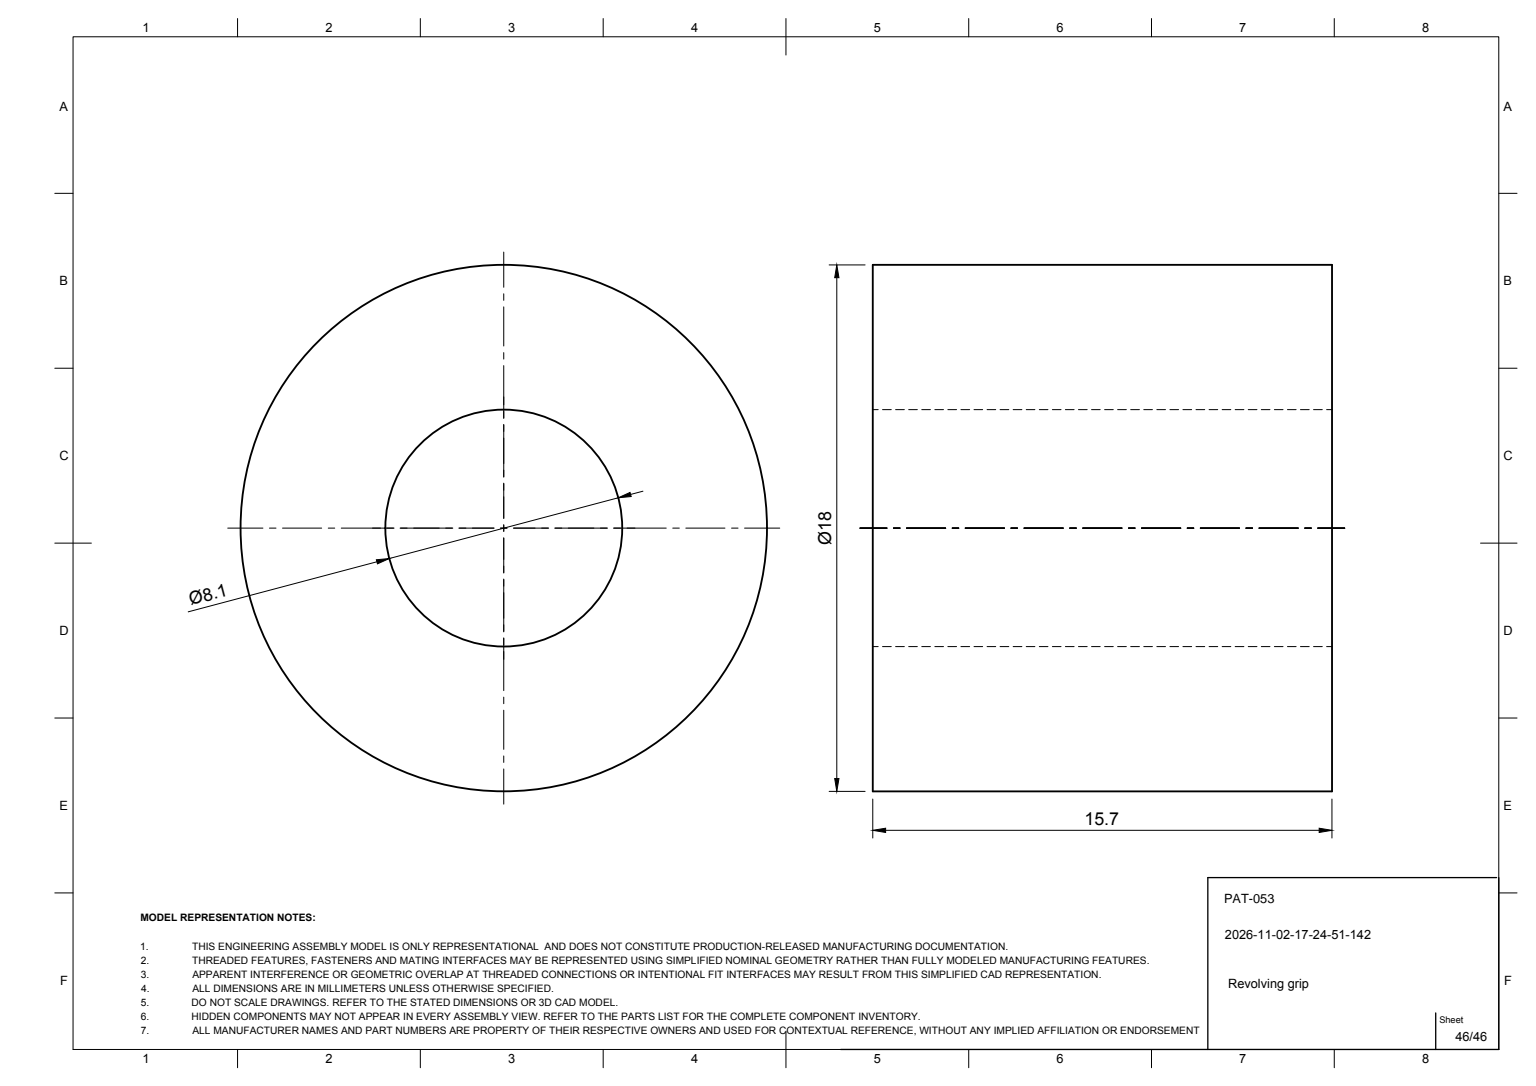
ISO-10303-21;
HEADER;
/* Generated by software containing ST-Developer
 * from STEP Tools, Inc. (www.steptools.com) 
 */

FILE_DESCRIPTION(
/* description */ ('Hand-operated arbor press'),
/* implementation_level */ '2;1');

FILE_NAME(
/* name */ 'Revolving grip.step',
/* time_stamp */ '2026-10-28T03:25:25-07:00',
/* author */ (''),
/* organization */ (''),
/* preprocessor_version */ 'ST-DEVELOPER v20.2',
/* originating_system */ 'Autodesk Translation Framework v15.17.0.0',
/* authorisation */ '');

FILE_SCHEMA (('AUTOMOTIVE_DESIGN { 1 0 10303 214 3 1 1 }'));
ENDSEC;

DATA;
#10=MECHANICAL_DESIGN_GEOMETRIC_PRESENTATION_REPRESENTATION('',(#634),#32751);
#543=SHAPE_REPRESENTATION_RELATIONSHIP('SRR','None',#32976,#585);
#585=ADVANCED_BREP_SHAPE_REPRESENTATION('',(#679),#32750);
#634=STYLED_ITEM('',(#33249),#679);
#679=MANIFOLD_SOLID_BREP('Body1',#12535);
#847=FACE_BOUND('',#2821,.T.);
#848=FACE_BOUND('',#2823,.T.);
#1291=PLANE('',#14148);
#1292=PLANE('',#14149);
#1970=FACE_OUTER_BOUND('',#2818,.T.);
#1971=FACE_OUTER_BOUND('',#2819,.T.);
#1972=FACE_OUTER_BOUND('',#2820,.T.);
#1973=FACE_OUTER_BOUND('',#2822,.T.);
#2818=EDGE_LOOP('',(#11630,#11631,#11632,#11633));
#2819=EDGE_LOOP('',(#11634,#11635,#11636,#11637));
#2820=EDGE_LOOP('',(#11638));
#2821=EDGE_LOOP('',(#11639));
#2822=EDGE_LOOP('',(#11640));
#2823=EDGE_LOOP('',(#11641));
#3993=LINE('',#32639,#5164);
#3994=LINE('',#32645,#5165);
#5164=VECTOR('',#17614,0.405);
#5165=VECTOR('',#17621,0.9);
#5552=CIRCLE('',#14143,0.405);
#5553=CIRCLE('',#14144,0.405);
#5554=CIRCLE('',#14146,0.9);
#5555=CIRCLE('',#14147,0.9);
#6661=VERTEX_POINT('',#32636);
#6662=VERTEX_POINT('',#32638);
#6663=VERTEX_POINT('',#32642);
#6664=VERTEX_POINT('',#32644);
#8318=EDGE_CURVE('',#6661,#6661,#5552,.T.);
#8319=EDGE_CURVE('',#6661,#6662,#3993,.T.);
#8320=EDGE_CURVE('',#6662,#6662,#5553,.T.);
#8321=EDGE_CURVE('',#6663,#6663,#5554,.T.);
#8322=EDGE_CURVE('',#6663,#6664,#3994,.T.);
#8323=EDGE_CURVE('',#6664,#6664,#5555,.T.);
#11630=ORIENTED_EDGE('',*,*,#8318,.F.);
#11631=ORIENTED_EDGE('',*,*,#8319,.T.);
#11632=ORIENTED_EDGE('',*,*,#8320,.T.);
#11633=ORIENTED_EDGE('',*,*,#8319,.F.);
#11634=ORIENTED_EDGE('',*,*,#8321,.F.);
#11635=ORIENTED_EDGE('',*,*,#8322,.T.);
#11636=ORIENTED_EDGE('',*,*,#8323,.T.);
#11637=ORIENTED_EDGE('',*,*,#8322,.F.);
#11638=ORIENTED_EDGE('',*,*,#8321,.T.);
#11639=ORIENTED_EDGE('',*,*,#8318,.T.);
#11640=ORIENTED_EDGE('',*,*,#8323,.F.);
#11641=ORIENTED_EDGE('',*,*,#8320,.F.);
#11800=CYLINDRICAL_SURFACE('',#14142,0.405);
#11801=CYLINDRICAL_SURFACE('',#14145,0.9);
#12479=ADVANCED_FACE('',(#1970),#11800,.F.);
#12480=ADVANCED_FACE('',(#1971),#11801,.T.);
#12481=ADVANCED_FACE('',(#1972,#847),#1291,.T.);
#12482=ADVANCED_FACE('',(#1973,#848),#1292,.F.);
#12535=CLOSED_SHELL('',(#12479,#12480,#12481,#12482));
#14141=AXIS2_PLACEMENT_3D('',#32634,#17608,#17609);
#14142=AXIS2_PLACEMENT_3D('',#32635,#17610,#17611);
#14143=AXIS2_PLACEMENT_3D('',#32637,#17612,#17613);
#14144=AXIS2_PLACEMENT_3D('',#32640,#17615,#17616);
#14145=AXIS2_PLACEMENT_3D('',#32641,#17617,#17618);
#14146=AXIS2_PLACEMENT_3D('',#32643,#17619,#17620);
#14147=AXIS2_PLACEMENT_3D('',#32646,#17622,#17623);
#14148=AXIS2_PLACEMENT_3D('',#32647,#17624,#17625);
#14149=AXIS2_PLACEMENT_3D('',#32648,#17626,#17627);
#17608=DIRECTION('axis',(0.,0.,1.));
#17609=DIRECTION('refdir',(1.,0.,0.));
#17610=DIRECTION('center_axis',(0.,1.,0.));
#17611=DIRECTION('ref_axis',(1.,0.,0.));
#17612=DIRECTION('center_axis',(0.,-1.,0.));
#17613=DIRECTION('ref_axis',(1.,0.,0.));
#17614=DIRECTION('',(0.,-1.,0.));
#17615=DIRECTION('center_axis',(0.,-1.,0.));
#17616=DIRECTION('ref_axis',(1.,0.,0.));
#17617=DIRECTION('center_axis',(0.,1.,0.));
#17618=DIRECTION('ref_axis',(1.,0.,0.));
#17619=DIRECTION('center_axis',(0.,1.,0.));
#17620=DIRECTION('ref_axis',(1.,0.,0.));
#17621=DIRECTION('',(0.,-1.,0.));
#17622=DIRECTION('center_axis',(0.,1.,0.));
#17623=DIRECTION('ref_axis',(1.,0.,0.));
#17624=DIRECTION('center_axis',(0.,1.,0.));
#17625=DIRECTION('ref_axis',(1.,0.,0.));
#17626=DIRECTION('center_axis',(0.,1.,0.));
#17627=DIRECTION('ref_axis',(1.,0.,0.));
#32634=CARTESIAN_POINT('',(0.,0.,0.));
#32635=CARTESIAN_POINT('Origin',(-3.25,6.8,29.));
#32636=CARTESIAN_POINT('',(-3.655,8.37,29.));
#32637=CARTESIAN_POINT('Origin',(-3.25,8.37,29.));
#32638=CARTESIAN_POINT('',(-3.655,6.8,29.));
#32639=CARTESIAN_POINT('',(-3.655,6.8,29.));
#32640=CARTESIAN_POINT('Origin',(-3.25,6.8,29.));
#32641=CARTESIAN_POINT('Origin',(-3.25,6.8,29.));
#32642=CARTESIAN_POINT('',(-4.15,8.37,29.));
#32643=CARTESIAN_POINT('Origin',(-3.25,8.37,29.));
#32644=CARTESIAN_POINT('',(-4.15,6.8,29.));
#32645=CARTESIAN_POINT('',(-4.15,6.8,29.));
#32646=CARTESIAN_POINT('Origin',(-3.25,6.8,29.));
#32647=CARTESIAN_POINT('Origin',(-3.25,8.37,29.));
#32648=CARTESIAN_POINT('Origin',(-3.25,6.8,29.));
#32701=UNCERTAINTY_MEASURE_WITH_UNIT(LENGTH_MEASURE(0.001),#32752,
'DISTANCE_ACCURACY_VALUE',
'Maximum model space distance between geometric entities at asserted c
onnectivities');
#32702=UNCERTAINTY_MEASURE_WITH_UNIT(LENGTH_MEASURE(0.001),#32752,
'DISTANCE_ACCURACY_VALUE',
'Maximum model space distance between geometric entities at asserted c
onnectivities');
#32750=(
GEOMETRIC_REPRESENTATION_CONTEXT(3)
GLOBAL_UNCERTAINTY_ASSIGNED_CONTEXT((#32701))
GLOBAL_UNIT_ASSIGNED_CONTEXT((#32752,#32754,#32755))
REPRESENTATION_CONTEXT('','3D')
);
#32751=(
GEOMETRIC_REPRESENTATION_CONTEXT(3)
GLOBAL_UNCERTAINTY_ASSIGNED_CONTEXT((#32702))
GLOBAL_UNIT_ASSIGNED_CONTEXT((#32752,#32754,#32755))
REPRESENTATION_CONTEXT('','3D')
);
#32752=(
LENGTH_UNIT()
NAMED_UNIT(*)
SI_UNIT(.CENTI.,.METRE.)
);
#32754=(
NAMED_UNIT(*)
PLANE_ANGLE_UNIT()
SI_UNIT($,.RADIAN.)
);
#32755=(
NAMED_UNIT(*)
SI_UNIT($,.STERADIAN.)
SOLID_ANGLE_UNIT()
);
#32803=SHAPE_DEFINITION_REPRESENTATION(#32923,#32976);
#32923=PRODUCT_DEFINITION_SHAPE('',$,#33025);
#32976=SHAPE_REPRESENTATION('',(#14141),#32750);
#32977=PRODUCT_DEFINITION_CONTEXT('part definition',#33123,'design');
#33025=PRODUCT_DEFINITION('Revolving grip','Revolving grip',#33073,#32977);
#33073=PRODUCT_DEFINITION_FORMATION('',$,#33172);
#33123=APPLICATION_CONTEXT(
'Core Data for Automotive Mechanical Design Process');
#33124=PRODUCT_CONTEXT('part definition',#33123,'mechanical');
#33172=PRODUCT('Revolving grip','Revolving grip','Revolving grip',(#33124));
#33243=COLOUR_RGB('Black',0.12,0.14,0.17);
#33244=FILL_AREA_STYLE_COLOUR('',#33243);
#33245=FILL_AREA_STYLE('',(#33244));
#33246=SURFACE_STYLE_FILL_AREA(#33245);
#33247=SURFACE_SIDE_STYLE('',(#33246));
#33248=SURFACE_STYLE_USAGE(.BOTH.,#33247);
#33249=PRESENTATION_STYLE_ASSIGNMENT((#33248));
ENDSEC;
END-ISO-10303-21;
